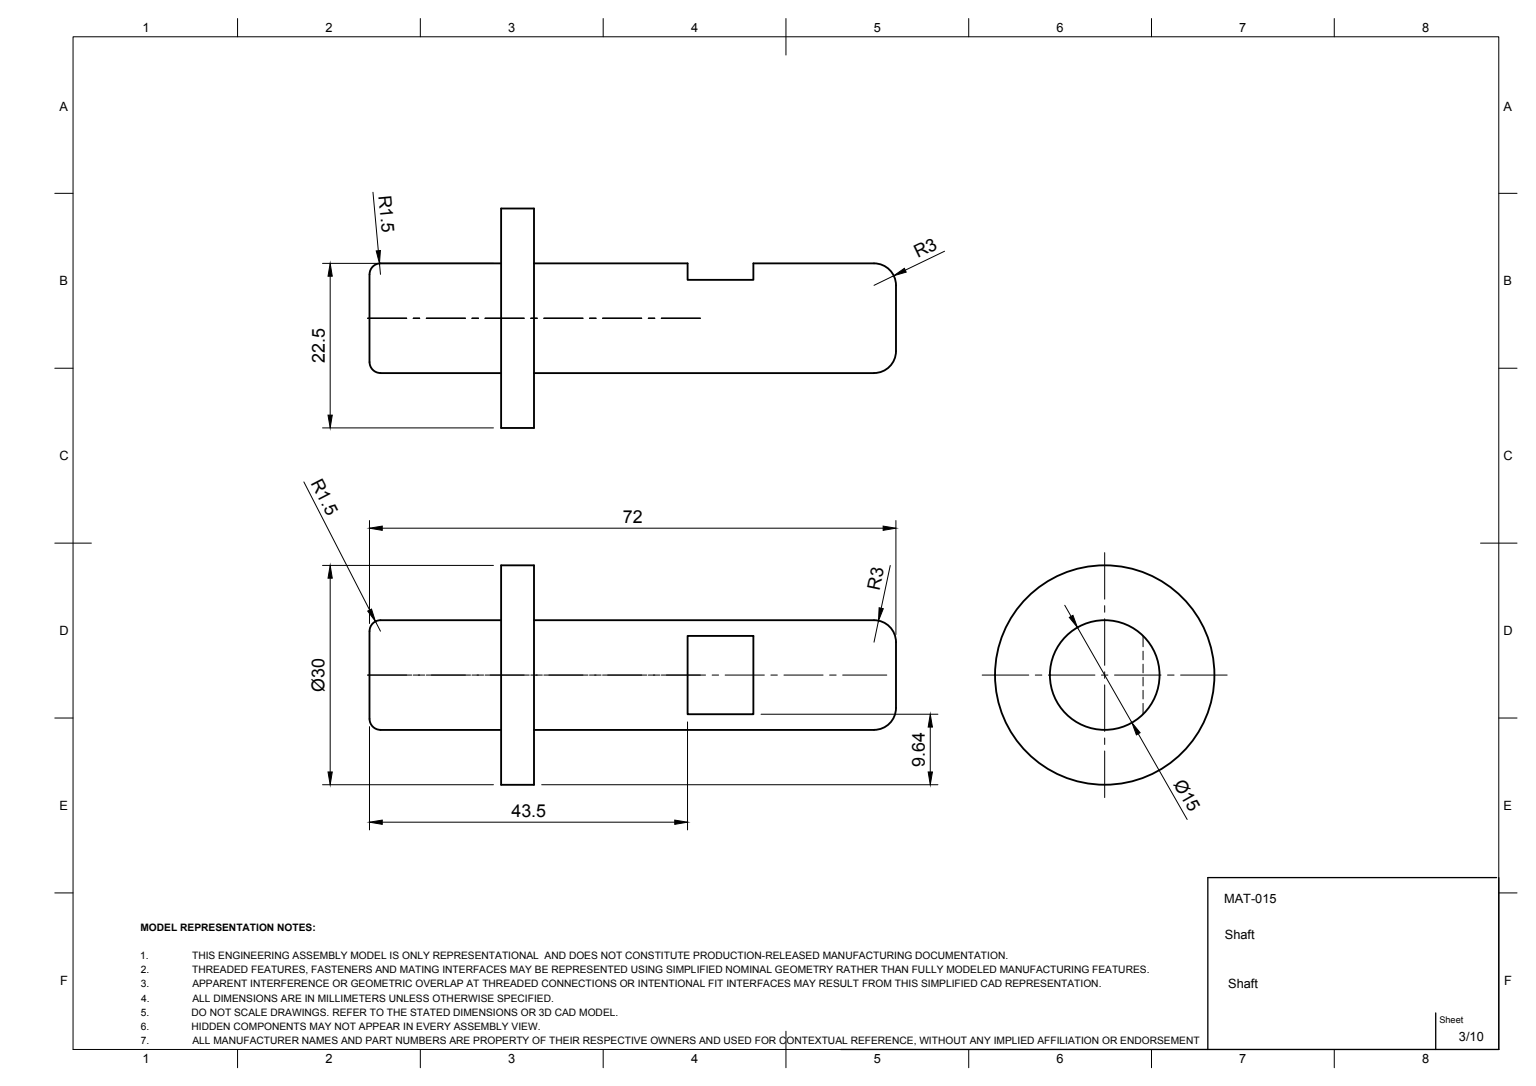
ISO-10303-21;
HEADER;
/* Generated by software containing ST-Developer
 * from STEP Tools, Inc. (www.steptools.com) 
 */

FILE_DESCRIPTION(
/* description */ ('STEP AP214'),
/* implementation_level */ '2;1');

FILE_NAME(
/* name */ 'Shaft.step',
/* time_stamp */ '2026-11-14T06:03:18-08:00',
/* author */ (''),
/* organization */ (''),
/* preprocessor_version */ 'ST-DEVELOPER v20.2',
/* originating_system */ 'Autodesk Translation Framework v15.17.0.0',
/* authorisation */ '');

FILE_SCHEMA (('AUTOMOTIVE_DESIGN { 1 0 10303 214 3 1 1 }'));
ENDSEC;

DATA;
#10=MECHANICAL_DESIGN_GEOMETRIC_PRESENTATION_REPRESENTATION('',(#72),#3206);
#56=SHAPE_REPRESENTATION_RELATIONSHIP('SRR','None',#3239,#64);
#64=ADVANCED_BREP_SHAPE_REPRESENTATION('',(#80),#3198);
#72=STYLED_ITEM('',(#3288),#80);
#80=MANIFOLD_SOLID_BREP('Body1',#1779);
#88=PLANE('',#1896);
#89=PLANE('',#1897);
#90=PLANE('',#1898);
#91=PLANE('',#1899);
#92=PLANE('',#1900);
#93=PLANE('',#1901);
#94=PLANE('',#1902);
#147=FACE_BOUND('',#617,.T.);
#148=FACE_BOUND('',#620,.T.);
#149=FACE_BOUND('',#622,.T.);
#188=LINE('',#2638,#333);
#189=LINE('',#2643,#334);
#190=LINE('',#2646,#335);
#191=LINE('',#2652,#336);
#192=LINE('',#2655,#337);
#193=LINE('',#2661,#338);
#194=LINE('',#2662,#339);
#333=VECTOR('',#2101,15.);
#334=VECTOR('',#2108,7.5);
#335=VECTOR('',#2111,7.49999999999999);
#336=VECTOR('',#2116,1000.);
#337=VECTOR('',#2119,1000.);
#338=VECTOR('',#2130,1000.);
#339=VECTOR('',#2131,1000.);
#478=CYLINDRICAL_SURFACE('',#1887,15.);
#479=CYLINDRICAL_SURFACE('',#1890,7.5);
#480=CYLINDRICAL_SURFACE('',#1892,7.49999999999999);
#512=FACE_OUTER_BOUND('',#612,.T.);
#513=FACE_OUTER_BOUND('',#613,.T.);
#514=FACE_OUTER_BOUND('',#614,.T.);
#515=FACE_OUTER_BOUND('',#615,.T.);
#516=FACE_OUTER_BOUND('',#616,.T.);
#517=FACE_OUTER_BOUND('',#618,.T.);
#518=FACE_OUTER_BOUND('',#619,.T.);
#519=FACE_OUTER_BOUND('',#621,.T.);
#520=FACE_OUTER_BOUND('',#623,.T.);
#521=FACE_OUTER_BOUND('',#624,.T.);
#522=FACE_OUTER_BOUND('',#625,.T.);
#523=FACE_OUTER_BOUND('',#626,.T.);
#612=EDGE_LOOP('',(#1217,#1218,#1219,#1220));
#613=EDGE_LOOP('',(#1221,#1222,#1223,#1224,#1225));
#614=EDGE_LOOP('',(#1226,#1227,#1228,#1229));
#615=EDGE_LOOP('',(#1230,#1231,#1232,#1233));
#616=EDGE_LOOP('',(#1234,#1235,#1236,#1237,#1238));
#617=EDGE_LOOP('',(#1239,#1240,#1241,#1242));
#618=EDGE_LOOP('',(#1243));
#619=EDGE_LOOP('',(#1244));
#620=EDGE_LOOP('',(#1245));
#621=EDGE_LOOP('',(#1246));
#622=EDGE_LOOP('',(#1247));
#623=EDGE_LOOP('',(#1248));
#624=EDGE_LOOP('',(#1249,#1250,#1251,#1252));
#625=EDGE_LOOP('',(#1253,#1254));
#626=EDGE_LOOP('',(#1255,#1256));
#753=CIRCLE('',#1879,7.5);
#754=CIRCLE('',#1880,1.5);
#755=CIRCLE('',#1881,6.);
#756=CIRCLE('',#1883,7.49999999999999);
#757=CIRCLE('',#1884,7.49999999999999);
#758=CIRCLE('',#1885,3.);
#759=CIRCLE('',#1886,4.49999999999999);
#760=CIRCLE('',#1888,15.);
#761=CIRCLE('',#1889,15.);
#762=CIRCLE('',#1891,7.5);
#763=CIRCLE('',#1893,7.5);
#764=CIRCLE('',#1894,7.49999999999999);
#765=CIRCLE('',#1895,7.49999999999999);
#834=VERTEX_POINT('',#2621);
#835=VERTEX_POINT('',#2623);
#836=VERTEX_POINT('',#2627);
#837=VERTEX_POINT('',#2628);
#838=VERTEX_POINT('',#2631);
#839=VERTEX_POINT('',#2635);
#840=VERTEX_POINT('',#2637);
#841=VERTEX_POINT('',#2641);
#842=VERTEX_POINT('',#2645);
#843=VERTEX_POINT('',#2648);
#844=VERTEX_POINT('',#2649);
#845=VERTEX_POINT('',#2651);
#846=VERTEX_POINT('',#2653);
#987=EDGE_CURVE('',#834,#834,#753,.T.);
#988=EDGE_CURVE('',#834,#835,#754,.T.);
#989=EDGE_CURVE('',#835,#835,#755,.T.);
#990=EDGE_CURVE('',#836,#837,#756,.T.);
#991=EDGE_CURVE('',#837,#836,#757,.T.);
#992=EDGE_CURVE('',#837,#838,#758,.T.);
#993=EDGE_CURVE('',#838,#838,#759,.T.);
#994=EDGE_CURVE('',#839,#839,#760,.T.);
#995=EDGE_CURVE('',#839,#840,#188,.T.);
#996=EDGE_CURVE('',#840,#840,#761,.T.);
#997=EDGE_CURVE('',#841,#841,#762,.T.);
#998=EDGE_CURVE('',#841,#834,#189,.T.);
#999=EDGE_CURVE('',#836,#842,#190,.T.);
#1000=EDGE_CURVE('',#842,#842,#763,.T.);
#1001=EDGE_CURVE('',#843,#844,#764,.T.);
#1002=EDGE_CURVE('',#843,#845,#191,.T.);
#1003=EDGE_CURVE('',#845,#846,#765,.T.);
#1004=EDGE_CURVE('',#846,#844,#192,.T.);
#1005=EDGE_CURVE('',#846,#845,#193,.T.);
#1006=EDGE_CURVE('',#844,#843,#194,.T.);
#1217=ORIENTED_EDGE('',*,*,#987,.F.);
#1218=ORIENTED_EDGE('',*,*,#988,.T.);
#1219=ORIENTED_EDGE('',*,*,#989,.F.);
#1220=ORIENTED_EDGE('',*,*,#988,.F.);
#1221=ORIENTED_EDGE('',*,*,#990,.F.);
#1222=ORIENTED_EDGE('',*,*,#991,.F.);
#1223=ORIENTED_EDGE('',*,*,#992,.T.);
#1224=ORIENTED_EDGE('',*,*,#993,.F.);
#1225=ORIENTED_EDGE('',*,*,#992,.F.);
#1226=ORIENTED_EDGE('',*,*,#994,.F.);
#1227=ORIENTED_EDGE('',*,*,#995,.T.);
#1228=ORIENTED_EDGE('',*,*,#996,.T.);
#1229=ORIENTED_EDGE('',*,*,#995,.F.);
#1230=ORIENTED_EDGE('',*,*,#997,.F.);
#1231=ORIENTED_EDGE('',*,*,#998,.T.);
#1232=ORIENTED_EDGE('',*,*,#987,.T.);
#1233=ORIENTED_EDGE('',*,*,#998,.F.);
#1234=ORIENTED_EDGE('',*,*,#990,.T.);
#1235=ORIENTED_EDGE('',*,*,#991,.T.);
#1236=ORIENTED_EDGE('',*,*,#999,.T.);
#1237=ORIENTED_EDGE('',*,*,#1000,.T.);
#1238=ORIENTED_EDGE('',*,*,#999,.F.);
#1239=ORIENTED_EDGE('',*,*,#1001,.F.);
#1240=ORIENTED_EDGE('',*,*,#1002,.T.);
#1241=ORIENTED_EDGE('',*,*,#1003,.T.);
#1242=ORIENTED_EDGE('',*,*,#1004,.T.);
#1243=ORIENTED_EDGE('',*,*,#989,.T.);
#1244=ORIENTED_EDGE('',*,*,#996,.F.);
#1245=ORIENTED_EDGE('',*,*,#997,.T.);
#1246=ORIENTED_EDGE('',*,*,#994,.T.);
#1247=ORIENTED_EDGE('',*,*,#1000,.F.);
#1248=ORIENTED_EDGE('',*,*,#993,.T.);
#1249=ORIENTED_EDGE('',*,*,#1005,.T.);
#1250=ORIENTED_EDGE('',*,*,#1002,.F.);
#1251=ORIENTED_EDGE('',*,*,#1006,.F.);
#1252=ORIENTED_EDGE('',*,*,#1004,.F.);
#1253=ORIENTED_EDGE('',*,*,#1006,.T.);
#1254=ORIENTED_EDGE('',*,*,#1001,.T.);
#1255=ORIENTED_EDGE('',*,*,#1005,.F.);
#1256=ORIENTED_EDGE('',*,*,#1003,.F.);
#1677=TOROIDAL_SURFACE('',#1878,6.,1.5);
#1678=TOROIDAL_SURFACE('',#1882,4.49999999999999,3.);
#1679=ADVANCED_FACE('',(#512),#1677,.T.);
#1680=ADVANCED_FACE('',(#513),#1678,.T.);
#1681=ADVANCED_FACE('',(#514),#478,.T.);
#1682=ADVANCED_FACE('',(#515),#479,.T.);
#1683=ADVANCED_FACE('',(#516,#147),#480,.T.);
#1684=ADVANCED_FACE('',(#517),#88,.F.);
#1685=ADVANCED_FACE('',(#518,#148),#89,.F.);
#1686=ADVANCED_FACE('',(#519,#149),#90,.F.);
#1687=ADVANCED_FACE('',(#520),#91,.F.);
#1688=ADVANCED_FACE('',(#521),#92,.F.);
#1689=ADVANCED_FACE('',(#522),#93,.T.);
#1690=ADVANCED_FACE('',(#523),#94,.F.);
#1779=CLOSED_SHELL('',(#1679,#1680,#1681,#1682,#1683,#1684,#1685,#1686,
#1687,#1688,#1689,#1690));
#1877=AXIS2_PLACEMENT_3D('',#2619,#2077,#2078);
#1878=AXIS2_PLACEMENT_3D('',#2620,#2079,#2080);
#1879=AXIS2_PLACEMENT_3D('',#2622,#2081,#2082);
#1880=AXIS2_PLACEMENT_3D('',#2624,#2083,#2084);
#1881=AXIS2_PLACEMENT_3D('',#2625,#2085,#2086);
#1882=AXIS2_PLACEMENT_3D('',#2626,#2087,#2088);
#1883=AXIS2_PLACEMENT_3D('',#2629,#2089,#2090);
#1884=AXIS2_PLACEMENT_3D('',#2630,#2091,#2092);
#1885=AXIS2_PLACEMENT_3D('',#2632,#2093,#2094);
#1886=AXIS2_PLACEMENT_3D('',#2633,#2095,#2096);
#1887=AXIS2_PLACEMENT_3D('',#2634,#2097,#2098);
#1888=AXIS2_PLACEMENT_3D('',#2636,#2099,#2100);
#1889=AXIS2_PLACEMENT_3D('',#2639,#2102,#2103);
#1890=AXIS2_PLACEMENT_3D('',#2640,#2104,#2105);
#1891=AXIS2_PLACEMENT_3D('',#2642,#2106,#2107);
#1892=AXIS2_PLACEMENT_3D('',#2644,#2109,#2110);
#1893=AXIS2_PLACEMENT_3D('',#2647,#2112,#2113);
#1894=AXIS2_PLACEMENT_3D('',#2650,#2114,#2115);
#1895=AXIS2_PLACEMENT_3D('',#2654,#2117,#2118);
#1896=AXIS2_PLACEMENT_3D('',#2656,#2120,#2121);
#1897=AXIS2_PLACEMENT_3D('',#2657,#2122,#2123);
#1898=AXIS2_PLACEMENT_3D('',#2658,#2124,#2125);
#1899=AXIS2_PLACEMENT_3D('',#2659,#2126,#2127);
#1900=AXIS2_PLACEMENT_3D('',#2660,#2128,#2129);
#1901=AXIS2_PLACEMENT_3D('',#2663,#2132,#2133);
#1902=AXIS2_PLACEMENT_3D('',#2664,#2134,#2135);
#2077=DIRECTION('axis',(0.,0.,1.));
#2078=DIRECTION('refdir',(1.,0.,0.));
#2079=DIRECTION('center_axis',(-1.,0.,0.));
#2080=DIRECTION('ref_axis',(0.,0.,1.));
#2081=DIRECTION('center_axis',(-1.,0.,0.));
#2082=DIRECTION('ref_axis',(0.,0.,1.));
#2083=DIRECTION('center_axis',(0.,-1.,1.22587125635694E-16));
#2084=DIRECTION('ref_axis',(0.,-1.22587125635694E-16,-1.));
#2085=DIRECTION('center_axis',(1.,0.,0.));
#2086=DIRECTION('ref_axis',(0.,0.,1.));
#2087=DIRECTION('center_axis',(1.,0.,0.));
#2088=DIRECTION('ref_axis',(0.,0.,-1.));
#2089=DIRECTION('center_axis',(1.,0.,0.));
#2090=DIRECTION('ref_axis',(0.,0.,-1.));
#2091=DIRECTION('center_axis',(1.,0.,0.));
#2092=DIRECTION('ref_axis',(0.,0.,-1.));
#2093=DIRECTION('center_axis',(0.,-1.,-1.22587125635694E-16));
#2094=DIRECTION('ref_axis',(0.,-1.22587125635694E-16,1.));
#2095=DIRECTION('center_axis',(-1.,0.,0.));
#2096=DIRECTION('ref_axis',(0.,0.,-1.));
#2097=DIRECTION('center_axis',(-1.,0.,0.));
#2098=DIRECTION('ref_axis',(0.,0.,1.));
#2099=DIRECTION('center_axis',(-1.,0.,0.));
#2100=DIRECTION('ref_axis',(0.,0.,1.));
#2101=DIRECTION('',(1.,0.,0.));
#2102=DIRECTION('center_axis',(-1.,0.,0.));
#2103=DIRECTION('ref_axis',(0.,0.,1.));
#2104=DIRECTION('center_axis',(-1.,0.,0.));
#2105=DIRECTION('ref_axis',(0.,0.,1.));
#2106=DIRECTION('center_axis',(-1.,0.,0.));
#2107=DIRECTION('ref_axis',(0.,0.,1.));
#2108=DIRECTION('',(1.,0.,0.));
#2109=DIRECTION('center_axis',(-1.,0.,0.));
#2110=DIRECTION('ref_axis',(0.,0.,1.));
#2111=DIRECTION('',(1.,0.,0.));
#2112=DIRECTION('center_axis',(-1.,0.,0.));
#2113=DIRECTION('ref_axis',(0.,0.,1.));
#2114=DIRECTION('center_axis',(1.,0.,0.));
#2115=DIRECTION('ref_axis',(0.,0.,-1.));
#2116=DIRECTION('',(1.,0.,0.));
#2117=DIRECTION('center_axis',(1.,0.,0.));
#2118=DIRECTION('ref_axis',(0.,0.,-1.));
#2119=DIRECTION('',(-1.,0.,0.));
#2120=DIRECTION('center_axis',(-1.,0.,0.));
#2121=DIRECTION('ref_axis',(0.,0.,1.));
#2122=DIRECTION('center_axis',(-1.,0.,0.));
#2123=DIRECTION('ref_axis',(0.,0.,1.));
#2124=DIRECTION('center_axis',(1.,0.,0.));
#2125=DIRECTION('ref_axis',(0.,0.,-1.));
#2126=DIRECTION('center_axis',(1.,0.,0.));
#2127=DIRECTION('ref_axis',(0.,0.,-1.));
#2128=DIRECTION('center_axis',(0.,-1.,0.));
#2129=DIRECTION('ref_axis',(0.,0.,-1.));
#2130=DIRECTION('',(0.,0.,-1.));
#2131=DIRECTION('',(0.,0.,-1.));
#2132=DIRECTION('center_axis',(1.,0.,0.));
#2133=DIRECTION('ref_axis',(0.,0.,-1.));
#2134=DIRECTION('center_axis',(1.,0.,0.));
#2135=DIRECTION('ref_axis',(0.,0.,-1.));
#2619=CARTESIAN_POINT('',(0.,0.,0.));
#2620=CARTESIAN_POINT('Origin',(9.56831985755466,0.0206871143368639,0.));
#2621=CARTESIAN_POINT('',(9.56831985755466,0.020687114336863,-7.5));
#2622=CARTESIAN_POINT('Origin',(9.56831985755466,0.0206871143368639,0.));
#2623=CARTESIAN_POINT('',(11.0683198575547,0.0206871143368632,-6.));
#2624=CARTESIAN_POINT('Origin',(9.56831985755466,0.0206871143368632,-6.));
#2625=CARTESIAN_POINT('Origin',(11.0683198575547,0.0206871143368639,0.));
#2626=CARTESIAN_POINT('Origin',(-57.9316801424454,0.0206871143368639,0.));
#2627=CARTESIAN_POINT('',(-57.9316801424454,0.0206871143368648,-7.49999999999999));
#2628=CARTESIAN_POINT('',(-57.9316801424454,0.020687114336863,7.49999999999999));
#2629=CARTESIAN_POINT('Origin',(-57.9316801424454,0.0206871143368639,0.));
#2630=CARTESIAN_POINT('Origin',(-57.9316801424454,0.0206871143368639,0.));
#2631=CARTESIAN_POINT('',(-60.9316801424454,0.0206871143368633,4.49999999999999));
#2632=CARTESIAN_POINT('Origin',(-57.9316801424454,0.0206871143368633,4.49999999999999));
#2633=CARTESIAN_POINT('Origin',(-60.9316801424454,0.0206871143368639,0.));
#2634=CARTESIAN_POINT('Origin',(-60.9316801424454,0.0206871143368639,0.));
#2635=CARTESIAN_POINT('',(-11.4316801424453,0.0206871143368621,-15.));
#2636=CARTESIAN_POINT('Origin',(-11.4316801424453,0.0206871143368639,0.));
#2637=CARTESIAN_POINT('',(-6.93168014244534,0.0206871143368621,-15.));
#2638=CARTESIAN_POINT('',(-60.9316801424454,0.0206871143368621,-15.));
#2639=CARTESIAN_POINT('Origin',(-6.93168014244534,0.0206871143368639,0.));
#2640=CARTESIAN_POINT('Origin',(-60.9316801424454,0.0206871143368639,0.));
#2641=CARTESIAN_POINT('',(-6.93168014244534,0.020687114336863,-7.5));
#2642=CARTESIAN_POINT('Origin',(-6.93168014244534,0.0206871143368639,0.));
#2643=CARTESIAN_POINT('',(-60.9316801424454,0.020687114336863,-7.5));
#2644=CARTESIAN_POINT('Origin',(-60.9316801424454,0.0206871143368639,0.));
#2645=CARTESIAN_POINT('',(-11.4316801424453,0.020687114336863,-7.49999999999999));
#2646=CARTESIAN_POINT('',(-60.9316801424454,0.020687114336863,-7.49999999999999));
#2647=CARTESIAN_POINT('Origin',(-11.4316801424453,0.0206871143368639,0.));
#2648=CARTESIAN_POINT('',(-41.4316801424454,5.27068711433686,-5.35607132140713));
#2649=CARTESIAN_POINT('',(-41.4316801424454,5.27068711433686,5.35607132140713));
#2650=CARTESIAN_POINT('Origin',(-41.4316801424454,0.0206871143368639,0.));
#2651=CARTESIAN_POINT('',(-32.4316801424454,5.27068711433686,-5.35607132140713));
#2652=CARTESIAN_POINT('',(-60.9316801424454,5.27068711433686,-5.35607132140713));
#2653=CARTESIAN_POINT('',(-32.4316801424454,5.27068711433686,5.35607132140713));
#2654=CARTESIAN_POINT('Origin',(-32.4316801424454,0.0206871143368639,0.));
#2655=CARTESIAN_POINT('',(-60.9316801424454,5.27068711433686,5.35607132140713));
#2656=CARTESIAN_POINT('Origin',(11.0683198575547,0.0206871143368639,0.));
#2657=CARTESIAN_POINT('Origin',(-6.93168014244535,7.52068711433686,0.));
#2658=CARTESIAN_POINT('Origin',(-11.4316801424453,15.0206871143369,0.));
#2659=CARTESIAN_POINT('Origin',(-60.9316801424454,7.52068711433686,0.));
#2660=CARTESIAN_POINT('Origin',(-41.4316801424454,5.27068711433686,0.));
#2661=CARTESIAN_POINT('',(-32.4316801424454,5.27068711433686,0.));
#2662=CARTESIAN_POINT('',(-41.4316801424454,5.27068711433686,5.84572916228895));
#2663=CARTESIAN_POINT('Origin',(-41.4316801424454,0.0206871143368639,0.));
#2664=CARTESIAN_POINT('Origin',(-32.4316801424454,0.0206871143368639,0.));
#3188=UNCERTAINTY_MEASURE_WITH_UNIT(LENGTH_MEASURE(0.01),#3207,
'DISTANCE_ACCURACY_VALUE',
'Maximum model space distance between geometric entities at asserted c
onnectivities');
#3196=UNCERTAINTY_MEASURE_WITH_UNIT(LENGTH_MEASURE(0.01),#3207,
'DISTANCE_ACCURACY_VALUE',
'Maximum model space distance between geometric entities at asserted c
onnectivities');
#3198=(
GEOMETRIC_REPRESENTATION_CONTEXT(3)
GLOBAL_UNCERTAINTY_ASSIGNED_CONTEXT((#3188))
GLOBAL_UNIT_ASSIGNED_CONTEXT((#3207,#3209,#3210))
REPRESENTATION_CONTEXT('','3D')
);
#3206=(
GEOMETRIC_REPRESENTATION_CONTEXT(3)
GLOBAL_UNCERTAINTY_ASSIGNED_CONTEXT((#3196))
GLOBAL_UNIT_ASSIGNED_CONTEXT((#3207,#3209,#3210))
REPRESENTATION_CONTEXT('','3D')
);
#3207=(
LENGTH_UNIT()
NAMED_UNIT(*)
SI_UNIT(.MILLI.,.METRE.)
);
#3209=(
NAMED_UNIT(*)
PLANE_ANGLE_UNIT()
SI_UNIT($,.RADIAN.)
);
#3210=(
NAMED_UNIT(*)
SI_UNIT($,.STERADIAN.)
SOLID_ANGLE_UNIT()
);
#3212=SHAPE_DEFINITION_REPRESENTATION(#3221,#3239);
#3221=PRODUCT_DEFINITION_SHAPE('',$,#3249);
#3239=SHAPE_REPRESENTATION('',(#1877),#3198);
#3247=PRODUCT_DEFINITION_CONTEXT('part definition',#3276,'design');
#3249=PRODUCT_DEFINITION('Shaft','Shaft',#3258,#3247);
#3258=PRODUCT_DEFINITION_FORMATION('',$,#3279);
#3276=APPLICATION_CONTEXT(
'Core Data for Automotive Mechanical Design Process');
#3277=PRODUCT_CONTEXT('part definition',#3276,'mechanical');
#3279=PRODUCT('Shaft','Shaft','Shaft',(#3277));
#3288=PRESENTATION_STYLE_ASSIGNMENT((#3292));
#3292=SURFACE_STYLE_USAGE(.BOTH.,#3296);
#3296=SURFACE_SIDE_STYLE('',(#3300));
#3300=SURFACE_STYLE_FILL_AREA(#3304);
#3304=FILL_AREA_STYLE('Opaque(61,176,222)',(#3308));
#3308=FILL_AREA_STYLE_COLOUR('Opaque(61,176,222)',#3312);
#3312=COLOUR_RGB('Opaque(61,176,222)',0.23921568627451,0.690196078431373,
0.870588235294118);
ENDSEC;
END-ISO-10303-21;
